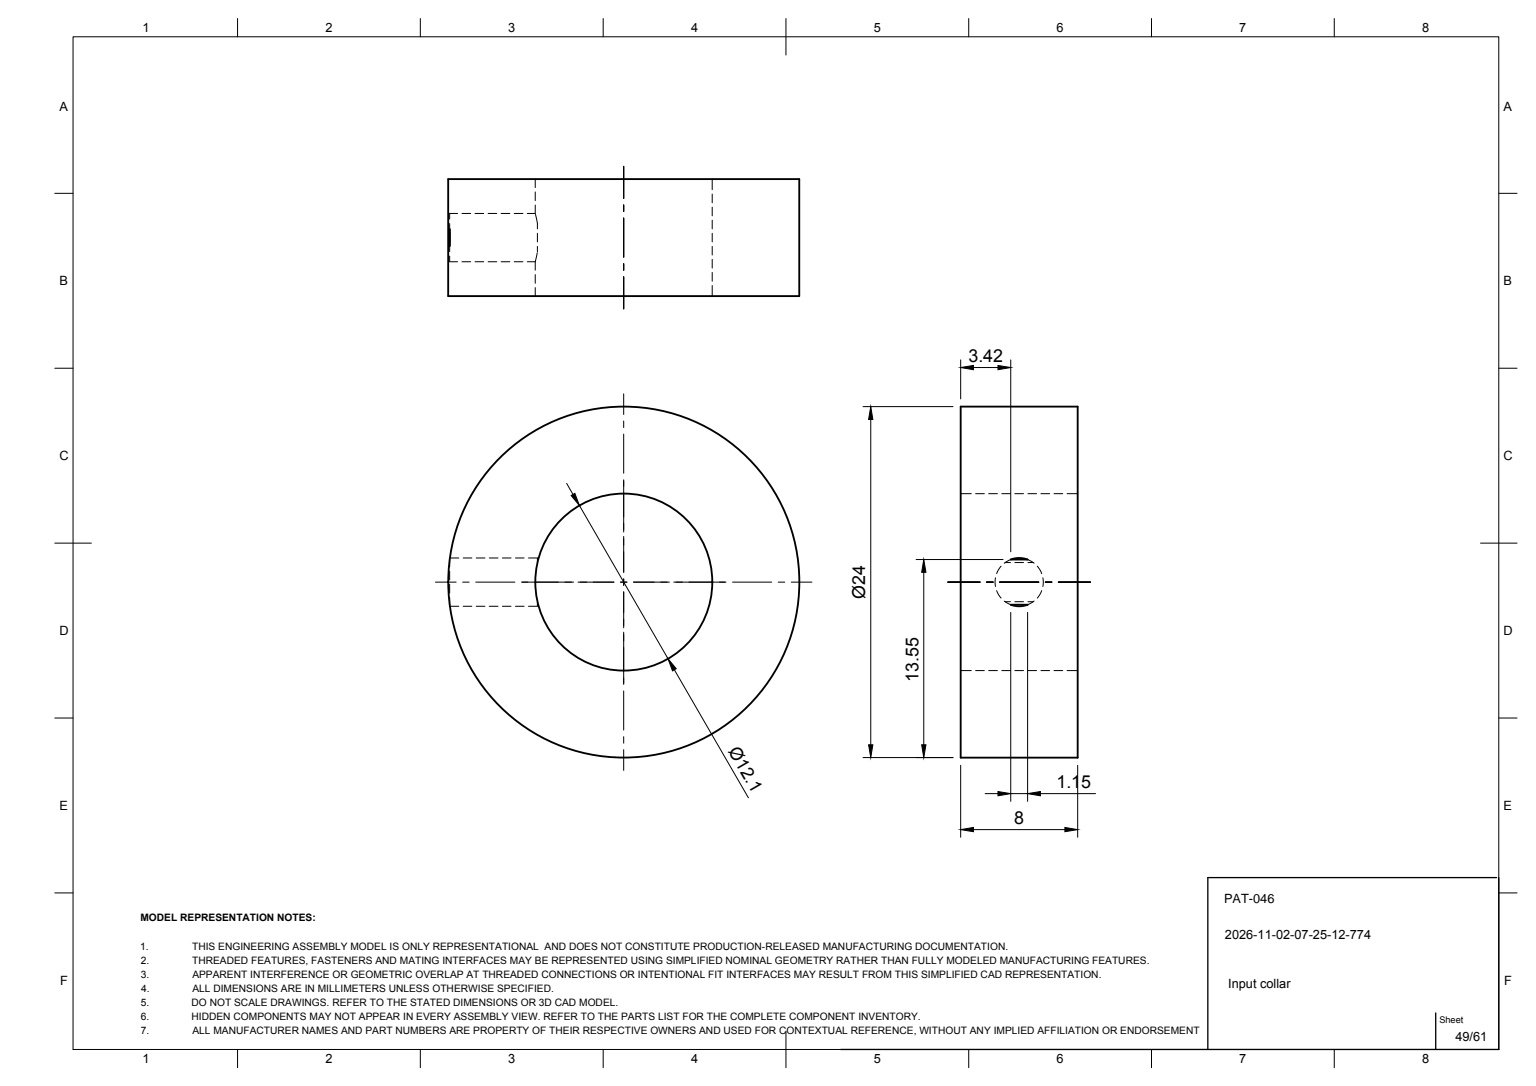
ISO-10303-21;
HEADER;
/* Generated by software containing ST-Developer
 * from STEP Tools, Inc. (www.steptools.com) 
 */

FILE_DESCRIPTION(
/* description */ ('Gear mesh backlash fixture'),
/* implementation_level */ '2;1');

FILE_NAME(
/* name */ 'Input collar.step',
/* time_stamp */ '2026-10-28T03:26:00-07:00',
/* author */ (''),
/* organization */ (''),
/* preprocessor_version */ 'ST-DEVELOPER v20.2',
/* originating_system */ 'Autodesk Translation Framework v15.17.0.0',
/* authorisation */ '');

FILE_SCHEMA (('AUTOMOTIVE_DESIGN { 1 0 10303 214 3 1 1 }'));
ENDSEC;

DATA;
#10=MECHANICAL_DESIGN_GEOMETRIC_PRESENTATION_REPRESENTATION('',(#1068),#57900);
#827=B_SPLINE_CURVE_WITH_KNOTS('',3,(#22118,#22119,#22120,#22121,#22122,
#22123,#22124,#22125,#22126,#22127,#22128,#22129,#22130,#22131),
 .UNSPECIFIED.,.F.,.F.,(4,2,2,2,2,2,4),(0.598759573717655,0.624973342427791,
0.687463163426144,0.749952984424497,0.812442805422849,0.874932626421202,
0.901146395131338),.UNSPECIFIED.);
#828=B_SPLINE_CURVE_WITH_KNOTS('',3,(#22135,#22136,#22137,#22138,#22139,
#22140,#22141,#22142),.UNSPECIFIED.,.F.,.F.,(4,2,2,4),(0.249984328141499,
0.312474149139851,0.374963970138204,0.40117773884834),.UNSPECIFIED.);
#829=B_SPLINE_CURVE_WITH_KNOTS('',3,(#22144,#22145,#22146,#22147,#22148,
#22149),.UNSPECIFIED.,.F.,.F.,(4,2,4),(0.441257277248191,0.497904393396855,
0.554551509545519),.UNSPECIFIED.);
#830=B_SPLINE_CURVE_WITH_KNOTS('',3,(#22150,#22151,#22152,#22153,#22154,
#22155,#22156),.UNSPECIFIED.,.F.,.F.,(4,3,4),(-0.0566471161400152,0.,0.0566471161486645),
 .UNSPECIFIED.);
#831=B_SPLINE_CURVE_WITH_KNOTS('',3,(#22157,#22158,#22159,#22160,#22161,
#22162,#22163,#22164),.UNSPECIFIED.,.F.,.F.,(4,2,2,4),(0.0987909174346573,
0.125004686144794,0.187494507143146,0.249984328141499),.UNSPECIFIED.);
#953=SHAPE_REPRESENTATION_RELATIONSHIP('SRR','None',#58153,#1003);
#1003=ADVANCED_BREP_SHAPE_REPRESENTATION('',(#1131),#57886);
#1068=STYLED_ITEM('',(#58479),#1131);
#1131=MANIFOLD_SOLID_BREP('Body1',#13630);
#1301=FACE_BOUND('',#3049,.T.);
#1302=FACE_BOUND('',#3051,.T.);
#1303=FACE_BOUND('',#3052,.T.);
#1304=FACE_BOUND('',#3054,.T.);
#1305=FACE_BOUND('',#3056,.T.);
#1565=PLANE('',#15095);
#1566=PLANE('',#15097);
#1567=PLANE('',#15103);
#1568=PLANE('',#15110);
#1569=PLANE('',#15111);
#2121=FACE_OUTER_BOUND('',#3044,.T.);
#2122=FACE_OUTER_BOUND('',#3045,.T.);
#2123=FACE_OUTER_BOUND('',#3046,.T.);
#2124=FACE_OUTER_BOUND('',#3047,.T.);
#2125=FACE_OUTER_BOUND('',#3048,.T.);
#2126=FACE_OUTER_BOUND('',#3050,.T.);
#2127=FACE_OUTER_BOUND('',#3053,.T.);
#2128=FACE_OUTER_BOUND('',#3055,.T.);
#3044=EDGE_LOOP('',(#10771,#10772));
#3045=EDGE_LOOP('',(#10773,#10774,#10775,#10776,#10777));
#3046=EDGE_LOOP('',(#10778,#10779,#10780,#10781,#10782,#10783,#10784,#10785,
#10786,#10787,#10788,#10789));
#3047=EDGE_LOOP('',(#10790,#10791));
#3048=EDGE_LOOP('',(#10792,#10793,#10794,#10795));
#3049=EDGE_LOOP('',(#10796,#10797,#10798,#10799,#10800));
#3050=EDGE_LOOP('',(#10801,#10802,#10803,#10804));
#3051=EDGE_LOOP('',(#10805,#10806));
#3052=EDGE_LOOP('',(#10807,#10808));
#3053=EDGE_LOOP('',(#10809));
#3054=EDGE_LOOP('',(#10810));
#3055=EDGE_LOOP('',(#10811));
#3056=EDGE_LOOP('',(#10812));
#3899=LINE('',#22103,#4788);
#3900=LINE('',#22108,#4789);
#3901=LINE('',#22114,#4790);
#3902=LINE('',#22143,#4791);
#3903=LINE('',#22166,#4792);
#3904=LINE('',#22171,#4793);
#3905=LINE('',#22177,#4794);
#4788=VECTOR('',#17868,1.);
#4789=VECTOR('',#17873,1.);
#4790=VECTOR('',#17878,1.);
#4791=VECTOR('',#17885,0.165);
#4792=VECTOR('',#17888,1.);
#4793=VECTOR('',#17893,0.605);
#4794=VECTOR('',#17900,1.2);
#5604=CIRCLE('',#15096,0.165);
#5605=CIRCLE('',#15098,0.165);
#5606=CIRCLE('',#15099,0.165);
#5607=CIRCLE('',#15100,0.165);
#5608=CIRCLE('',#15102,0.165);
#5609=CIRCLE('',#15105,0.605);
#5610=CIRCLE('',#15106,0.605);
#5611=CIRCLE('',#15108,1.2);
#5612=CIRCLE('',#15109,1.2);
#6422=VERTEX_POINT('',#22101);
#6423=VERTEX_POINT('',#22102);
#6424=VERTEX_POINT('',#22106);
#6425=VERTEX_POINT('',#22107);
#6426=VERTEX_POINT('',#22109);
#6427=VERTEX_POINT('',#22111);
#6428=VERTEX_POINT('',#22113);
#6429=VERTEX_POINT('',#22117);
#6430=VERTEX_POINT('',#22132);
#6431=VERTEX_POINT('',#22134);
#6432=VERTEX_POINT('',#22168);
#6433=VERTEX_POINT('',#22170);
#6434=VERTEX_POINT('',#22174);
#6435=VERTEX_POINT('',#22176);
#7972=EDGE_CURVE('',#6422,#6423,#3899,.T.);
#7973=EDGE_CURVE('',#6422,#6423,#5604,.T.);
#7974=EDGE_CURVE('',#6424,#6425,#3900,.T.);
#7975=EDGE_CURVE('',#6426,#6424,#5605,.T.);
#7976=EDGE_CURVE('',#6427,#6426,#5606,.T.);
#7977=EDGE_CURVE('',#6428,#6427,#3901,.T.);
#7978=EDGE_CURVE('',#6425,#6428,#5607,.T.);
#7979=EDGE_CURVE('',#6429,#6422,#827,.T.);
#7980=EDGE_CURVE('',#6430,#6429,#5608,.T.);
#7981=EDGE_CURVE('',#6431,#6430,#828,.T.);
#7982=EDGE_CURVE('',#6431,#6426,#3902,.T.);
#7983=EDGE_CURVE('',#6425,#6424,#829,.T.);
#7984=EDGE_CURVE('',#6427,#6428,#830,.T.);
#7985=EDGE_CURVE('',#6423,#6431,#831,.T.);
#7986=EDGE_CURVE('',#6430,#6429,#3903,.T.);
#7987=EDGE_CURVE('',#6432,#6432,#5609,.T.);
#7988=EDGE_CURVE('',#6432,#6433,#3904,.T.);
#7989=EDGE_CURVE('',#6433,#6433,#5610,.T.);
#7990=EDGE_CURVE('',#6434,#6434,#5611,.T.);
#7991=EDGE_CURVE('',#6434,#6435,#3905,.T.);
#7992=EDGE_CURVE('',#6435,#6435,#5612,.T.);
#10771=ORIENTED_EDGE('',*,*,#7972,.F.);
#10772=ORIENTED_EDGE('',*,*,#7973,.T.);
#10773=ORIENTED_EDGE('',*,*,#7974,.F.);
#10774=ORIENTED_EDGE('',*,*,#7975,.F.);
#10775=ORIENTED_EDGE('',*,*,#7976,.F.);
#10776=ORIENTED_EDGE('',*,*,#7977,.F.);
#10777=ORIENTED_EDGE('',*,*,#7978,.F.);
#10778=ORIENTED_EDGE('',*,*,#7979,.F.);
#10779=ORIENTED_EDGE('',*,*,#7980,.F.);
#10780=ORIENTED_EDGE('',*,*,#7981,.F.);
#10781=ORIENTED_EDGE('',*,*,#7982,.T.);
#10782=ORIENTED_EDGE('',*,*,#7975,.T.);
#10783=ORIENTED_EDGE('',*,*,#7983,.F.);
#10784=ORIENTED_EDGE('',*,*,#7978,.T.);
#10785=ORIENTED_EDGE('',*,*,#7984,.F.);
#10786=ORIENTED_EDGE('',*,*,#7976,.T.);
#10787=ORIENTED_EDGE('',*,*,#7982,.F.);
#10788=ORIENTED_EDGE('',*,*,#7985,.F.);
#10789=ORIENTED_EDGE('',*,*,#7973,.F.);
#10790=ORIENTED_EDGE('',*,*,#7986,.F.);
#10791=ORIENTED_EDGE('',*,*,#7980,.T.);
#10792=ORIENTED_EDGE('',*,*,#7987,.F.);
#10793=ORIENTED_EDGE('',*,*,#7988,.T.);
#10794=ORIENTED_EDGE('',*,*,#7989,.T.);
#10795=ORIENTED_EDGE('',*,*,#7988,.F.);
#10796=ORIENTED_EDGE('',*,*,#7985,.T.);
#10797=ORIENTED_EDGE('',*,*,#7981,.T.);
#10798=ORIENTED_EDGE('',*,*,#7986,.T.);
#10799=ORIENTED_EDGE('',*,*,#7979,.T.);
#10800=ORIENTED_EDGE('',*,*,#7972,.T.);
#10801=ORIENTED_EDGE('',*,*,#7990,.F.);
#10802=ORIENTED_EDGE('',*,*,#7991,.T.);
#10803=ORIENTED_EDGE('',*,*,#7992,.T.);
#10804=ORIENTED_EDGE('',*,*,#7991,.F.);
#10805=ORIENTED_EDGE('',*,*,#7983,.T.);
#10806=ORIENTED_EDGE('',*,*,#7974,.T.);
#10807=ORIENTED_EDGE('',*,*,#7984,.T.);
#10808=ORIENTED_EDGE('',*,*,#7977,.T.);
#10809=ORIENTED_EDGE('',*,*,#7990,.T.);
#10810=ORIENTED_EDGE('',*,*,#7987,.T.);
#10811=ORIENTED_EDGE('',*,*,#7992,.F.);
#10812=ORIENTED_EDGE('',*,*,#7989,.F.);
#12726=CYLINDRICAL_SURFACE('',#15101,0.165);
#12727=CYLINDRICAL_SURFACE('',#15104,0.605);
#12728=CYLINDRICAL_SURFACE('',#15107,1.2);
#13238=ADVANCED_FACE('',(#2121),#1565,.T.);
#13239=ADVANCED_FACE('',(#2122),#1566,.F.);
#13240=ADVANCED_FACE('',(#2123),#12726,.F.);
#13241=ADVANCED_FACE('',(#2124),#1567,.T.);
#13242=ADVANCED_FACE('',(#2125,#1301),#12727,.F.);
#13243=ADVANCED_FACE('',(#2126,#1302,#1303),#12728,.T.);
#13244=ADVANCED_FACE('',(#2127,#1304),#1568,.T.);
#13245=ADVANCED_FACE('',(#2128,#1305),#1569,.F.);
#13630=CLOSED_SHELL('',(#13238,#13239,#13240,#13241,#13242,#13243,#13244,
#13245));
#15094=AXIS2_PLACEMENT_3D('',#22099,#17864,#17865);
#15095=AXIS2_PLACEMENT_3D('',#22100,#17866,#17867);
#15096=AXIS2_PLACEMENT_3D('',#22104,#17869,#17870);
#15097=AXIS2_PLACEMENT_3D('',#22105,#17871,#17872);
#15098=AXIS2_PLACEMENT_3D('',#22110,#17874,#17875);
#15099=AXIS2_PLACEMENT_3D('',#22112,#17876,#17877);
#15100=AXIS2_PLACEMENT_3D('',#22115,#17879,#17880);
#15101=AXIS2_PLACEMENT_3D('',#22116,#17881,#17882);
#15102=AXIS2_PLACEMENT_3D('',#22133,#17883,#17884);
#15103=AXIS2_PLACEMENT_3D('',#22165,#17886,#17887);
#15104=AXIS2_PLACEMENT_3D('',#22167,#17889,#17890);
#15105=AXIS2_PLACEMENT_3D('',#22169,#17891,#17892);
#15106=AXIS2_PLACEMENT_3D('',#22172,#17894,#17895);
#15107=AXIS2_PLACEMENT_3D('',#22173,#17896,#17897);
#15108=AXIS2_PLACEMENT_3D('',#22175,#17898,#17899);
#15109=AXIS2_PLACEMENT_3D('',#22178,#17901,#17902);
#15110=AXIS2_PLACEMENT_3D('',#22179,#17903,#17904);
#15111=AXIS2_PLACEMENT_3D('',#22180,#17905,#17906);
#17864=DIRECTION('axis',(0.,0.,1.));
#17865=DIRECTION('refdir',(1.,0.,0.));
#17866=DIRECTION('center_axis',(1.,0.,0.));
#17867=DIRECTION('ref_axis',(0.,0.,-1.));
#17868=DIRECTION('',(0.,0.,1.));
#17869=DIRECTION('center_axis',(1.,0.,0.));
#17870=DIRECTION('ref_axis',(0.,0.,-1.));
#17871=DIRECTION('center_axis',(1.,0.,0.));
#17872=DIRECTION('ref_axis',(0.,0.,-1.));
#17873=DIRECTION('',(0.,0.,-1.));
#17874=DIRECTION('center_axis',(1.,0.,0.));
#17875=DIRECTION('ref_axis',(0.,0.,-1.));
#17876=DIRECTION('center_axis',(1.,0.,0.));
#17877=DIRECTION('ref_axis',(0.,0.,-1.));
#17878=DIRECTION('',(0.,0.,1.));
#17879=DIRECTION('center_axis',(1.,0.,0.));
#17880=DIRECTION('ref_axis',(0.,0.,-1.));
#17881=DIRECTION('center_axis',(1.,0.,0.));
#17882=DIRECTION('ref_axis',(0.,0.,-1.));
#17883=DIRECTION('center_axis',(1.,0.,0.));
#17884=DIRECTION('ref_axis',(0.,0.,-1.));
#17885=DIRECTION('',(1.,0.,0.));
#17886=DIRECTION('center_axis',(1.,0.,0.));
#17887=DIRECTION('ref_axis',(0.,0.,-1.));
#17888=DIRECTION('',(0.,0.,-1.));
#17889=DIRECTION('center_axis',(0.,0.,1.));
#17890=DIRECTION('ref_axis',(1.,0.,0.));
#17891=DIRECTION('center_axis',(0.,0.,-1.));
#17892=DIRECTION('ref_axis',(1.,0.,0.));
#17893=DIRECTION('',(0.,0.,-1.));
#17894=DIRECTION('center_axis',(0.,0.,-1.));
#17895=DIRECTION('ref_axis',(1.,0.,0.));
#17896=DIRECTION('center_axis',(0.,0.,1.));
#17897=DIRECTION('ref_axis',(1.,0.,0.));
#17898=DIRECTION('center_axis',(0.,0.,1.));
#17899=DIRECTION('ref_axis',(1.,0.,0.));
#17900=DIRECTION('',(0.,0.,-1.));
#17901=DIRECTION('center_axis',(0.,0.,1.));
#17902=DIRECTION('ref_axis',(1.,0.,0.));
#17903=DIRECTION('center_axis',(0.,0.,1.));
#17904=DIRECTION('ref_axis',(1.,0.,0.));
#17905=DIRECTION('center_axis',(0.,0.,1.));
#17906=DIRECTION('ref_axis',(1.,0.,0.));
#22099=CARTESIAN_POINT('',(0.,0.,0.));
#22100=CARTESIAN_POINT('Origin',(0.59,0.,5.4));
#22101=CARTESIAN_POINT('',(0.59,0.133884278389959,5.30356349239007));
#22102=CARTESIAN_POINT('',(0.59,0.133884278389959,5.49643650760993));
#22103=CARTESIAN_POINT('',(0.59,0.133884278389959,5.));
#22104=CARTESIAN_POINT('Origin',(0.59,0.,5.4));
#22105=CARTESIAN_POINT('Origin',(1.19,0.,5.4));
#22106=CARTESIAN_POINT('',(1.19,-0.154596248337402,5.45766281297336));
#22107=CARTESIAN_POINT('',(1.19,-0.154596248337402,5.34233718702664));
#22108=CARTESIAN_POINT('',(1.19,-0.154596248337402,5.));
#22109=CARTESIAN_POINT('',(1.19,-2.02066721859313E-17,5.565));
#22110=CARTESIAN_POINT('Origin',(1.19,0.,5.4));
#22111=CARTESIAN_POINT('',(1.19,0.154596248337402,5.45766281297336));
#22112=CARTESIAN_POINT('Origin',(1.19,0.,5.4));
#22113=CARTESIAN_POINT('',(1.19,0.154596248337402,5.34233718702664));
#22114=CARTESIAN_POINT('',(1.19,0.154596248337402,5.));
#22115=CARTESIAN_POINT('Origin',(1.19,0.,5.4));
#22116=CARTESIAN_POINT('Origin',(0.59,0.,5.4));
#22117=CARTESIAN_POINT('',(0.59,-0.133884278389959,5.30356349239007));
#22118=CARTESIAN_POINT('Ctrl Pts',(0.59,-0.133884278389959,5.30356349239007));
#22119=CARTESIAN_POINT('Ctrl Pts',(0.591198403406107,-0.128603165341393,
5.29623164237676));
#22120=CARTESIAN_POINT('Ctrl Pts',(0.59244064128815,-0.122792448979943,
5.28944721118838));
#22121=CARTESIAN_POINT('Ctrl Pts',(0.596510641114135,-0.10208383195986,
5.2687385941683));
#22122=CARTESIAN_POINT('Ctrl Pts',(0.599544094983168,-0.0836002135946608,
5.2560565239921));
#22123=CARTESIAN_POINT('Ctrl Pts',(0.603817074382984,-0.0429774150042653,
5.23918438436621));
#22124=CARTESIAN_POINT('Ctrl Pts',(0.605,-0.0208299403327843,5.235));
#22125=CARTESIAN_POINT('Ctrl Pts',(0.605,0.0208299403327842,5.235));
#22126=CARTESIAN_POINT('Ctrl Pts',(0.603817074382984,0.0429774150042653,
5.23918438436621));
#22127=CARTESIAN_POINT('Ctrl Pts',(0.599544094983168,0.0836002135946608,
5.2560565239921));
#22128=CARTESIAN_POINT('Ctrl Pts',(0.596510641114135,0.10208383195986,5.2687385941683));
#22129=CARTESIAN_POINT('Ctrl Pts',(0.59244064128815,0.122792448979943,5.28944721118838));
#22130=CARTESIAN_POINT('Ctrl Pts',(0.591198403406107,0.128603165341393,
5.29623164237676));
#22131=CARTESIAN_POINT('Ctrl Pts',(0.59,0.133884278389959,5.30356349239007));
#22132=CARTESIAN_POINT('',(0.59,-0.133884278389959,5.49643650760993));
#22133=CARTESIAN_POINT('Origin',(0.59,0.,5.4));
#22134=CARTESIAN_POINT('',(0.605,2.8060580378524E-17,5.565));
#22135=CARTESIAN_POINT('Ctrl Pts',(0.605,7.63278329429795E-17,5.565));
#22136=CARTESIAN_POINT('Ctrl Pts',(0.605,-0.0208299403327841,5.565));
#22137=CARTESIAN_POINT('Ctrl Pts',(0.603817074382984,-0.0429774150042653,
5.5608156156338));
#22138=CARTESIAN_POINT('Ctrl Pts',(0.599544094983168,-0.0836002135946608,
5.5439434760079));
#22139=CARTESIAN_POINT('Ctrl Pts',(0.596510641114135,-0.10208383195986,
5.5312614058317));
#22140=CARTESIAN_POINT('Ctrl Pts',(0.59244064128815,-0.122792448979943,
5.51055278881162));
#22141=CARTESIAN_POINT('Ctrl Pts',(0.591198403406107,-0.128603165341393,
5.50376835762324));
#22142=CARTESIAN_POINT('Ctrl Pts',(0.59,-0.133884278389959,5.49643650760993));
#22143=CARTESIAN_POINT('',(0.59,-2.02066721859313E-17,5.565));
#22144=CARTESIAN_POINT('Ctrl Pts',(1.19,-0.154596248337401,5.34233718702664));
#22145=CARTESIAN_POINT('Ctrl Pts',(1.18909117046716,-0.161591936497431,
5.36109289956149));
#22146=CARTESIAN_POINT('Ctrl Pts',(1.18860212013945,-0.165,5.38111762795045));
#22147=CARTESIAN_POINT('Ctrl Pts',(1.18860212013945,-0.165,5.41888237204955));
#22148=CARTESIAN_POINT('Ctrl Pts',(1.18909117046716,-0.161591936497431,
5.43890710043851));
#22149=CARTESIAN_POINT('Ctrl Pts',(1.19,-0.154596248337402,5.45766281297336));
#22150=CARTESIAN_POINT('Ctrl Pts',(1.19,0.154596248337402,5.45766281297336));
#22151=CARTESIAN_POINT('Ctrl Pts',(1.18909117046841,0.161591936487821,5.43890710046428));
#22152=CARTESIAN_POINT('Ctrl Pts',(1.18860212013945,0.165,5.41888237204667));
#22153=CARTESIAN_POINT('Ctrl Pts',(1.18860212013945,0.165,5.4));
#22154=CARTESIAN_POINT('Ctrl Pts',(1.18860212013945,0.165,5.38111762795045));
#22155=CARTESIAN_POINT('Ctrl Pts',(1.18909117046716,0.161591936497431,5.36109289956149));
#22156=CARTESIAN_POINT('Ctrl Pts',(1.19,0.154596248337401,5.34233718702664));
#22157=CARTESIAN_POINT('Ctrl Pts',(0.59,0.133884278389959,5.49643650760993));
#22158=CARTESIAN_POINT('Ctrl Pts',(0.591198403406107,0.128603165341393,
5.50376835762324));
#22159=CARTESIAN_POINT('Ctrl Pts',(0.59244064128815,0.122792448979943,5.51055278881162));
#22160=CARTESIAN_POINT('Ctrl Pts',(0.596510641114135,0.10208383195986,5.5312614058317));
#22161=CARTESIAN_POINT('Ctrl Pts',(0.599544094983168,0.0836002135946608,
5.5439434760079));
#22162=CARTESIAN_POINT('Ctrl Pts',(0.603817074382984,0.0429774150042653,
5.5608156156338));
#22163=CARTESIAN_POINT('Ctrl Pts',(0.605,0.0208299403327841,5.565));
#22164=CARTESIAN_POINT('Ctrl Pts',(0.605,-7.63278329429795E-17,5.565));
#22165=CARTESIAN_POINT('Origin',(0.59,0.,5.4));
#22166=CARTESIAN_POINT('',(0.59,-0.133884278389959,5.));
#22167=CARTESIAN_POINT('Origin',(0.,0.,5.));
#22168=CARTESIAN_POINT('',(-0.605,-7.40911313484149E-17,5.8));
#22169=CARTESIAN_POINT('Origin',(0.,0.,5.8));
#22170=CARTESIAN_POINT('',(-0.605,-7.40911313484149E-17,5.));
#22171=CARTESIAN_POINT('',(-0.605,-7.40911313484149E-17,5.));
#22172=CARTESIAN_POINT('Origin',(0.,0.,5.));
#22173=CARTESIAN_POINT('Origin',(0.,0.,5.));
#22174=CARTESIAN_POINT('',(-1.2,-1.46957615897682E-16,5.8));
#22175=CARTESIAN_POINT('Origin',(0.,0.,5.8));
#22176=CARTESIAN_POINT('',(-1.2,-1.46957615897682E-16,5.));
#22177=CARTESIAN_POINT('',(-1.2,-1.46957615897682E-16,5.));
#22178=CARTESIAN_POINT('Origin',(0.,0.,5.));
#22179=CARTESIAN_POINT('Origin',(0.,0.,5.8));
#22180=CARTESIAN_POINT('Origin',(0.,0.,5.));
#57827=UNCERTAINTY_MEASURE_WITH_UNIT(LENGTH_MEASURE(0.001),#57901,
'DISTANCE_ACCURACY_VALUE',
'Maximum model space distance between geometric entities at asserted c
onnectivities');
#57841=UNCERTAINTY_MEASURE_WITH_UNIT(LENGTH_MEASURE(0.001),#57901,
'DISTANCE_ACCURACY_VALUE',
'Maximum model space distance between geometric entities at asserted c
onnectivities');
#57886=(
GEOMETRIC_REPRESENTATION_CONTEXT(3)
GLOBAL_UNCERTAINTY_ASSIGNED_CONTEXT((#57827))
GLOBAL_UNIT_ASSIGNED_CONTEXT((#57901,#57903,#57904))
REPRESENTATION_CONTEXT('','3D')
);
#57900=(
GEOMETRIC_REPRESENTATION_CONTEXT(3)
GLOBAL_UNCERTAINTY_ASSIGNED_CONTEXT((#57841))
GLOBAL_UNIT_ASSIGNED_CONTEXT((#57901,#57903,#57904))
REPRESENTATION_CONTEXT('','3D')
);
#57901=(
LENGTH_UNIT()
NAMED_UNIT(*)
SI_UNIT(.CENTI.,.METRE.)
);
#57903=(
NAMED_UNIT(*)
PLANE_ANGLE_UNIT()
SI_UNIT($,.RADIAN.)
);
#57904=(
NAMED_UNIT(*)
SI_UNIT($,.STERADIAN.)
SOLID_ANGLE_UNIT()
);
#57949=SHAPE_DEFINITION_REPRESENTATION(#58020,#58153);
#58020=PRODUCT_DEFINITION_SHAPE('',$,#58212);
#58153=SHAPE_REPRESENTATION('',(#15094),#57886);
#58167=PRODUCT_DEFINITION_CONTEXT('part definition',#58343,'design');
#58212=PRODUCT_DEFINITION('Input collar','Input collar',#58270,#58167);
#58270=PRODUCT_DEFINITION_FORMATION('',$,#58389);
#58343=APPLICATION_CONTEXT(
'Core Data for Automotive Mechanical Design Process');
#58344=PRODUCT_CONTEXT('part definition',#58343,'mechanical');
#58389=PRODUCT('Input collar','Input collar','Input collar',(#58344));
#58473=COLOUR_RGB('Off White',0.89,0.88,0.83);
#58474=FILL_AREA_STYLE_COLOUR('',#58473);
#58475=FILL_AREA_STYLE('',(#58474));
#58476=SURFACE_STYLE_FILL_AREA(#58475);
#58477=SURFACE_SIDE_STYLE('',(#58476));
#58478=SURFACE_STYLE_USAGE(.BOTH.,#58477);
#58479=PRESENTATION_STYLE_ASSIGNMENT((#58478));
ENDSEC;
END-ISO-10303-21;
